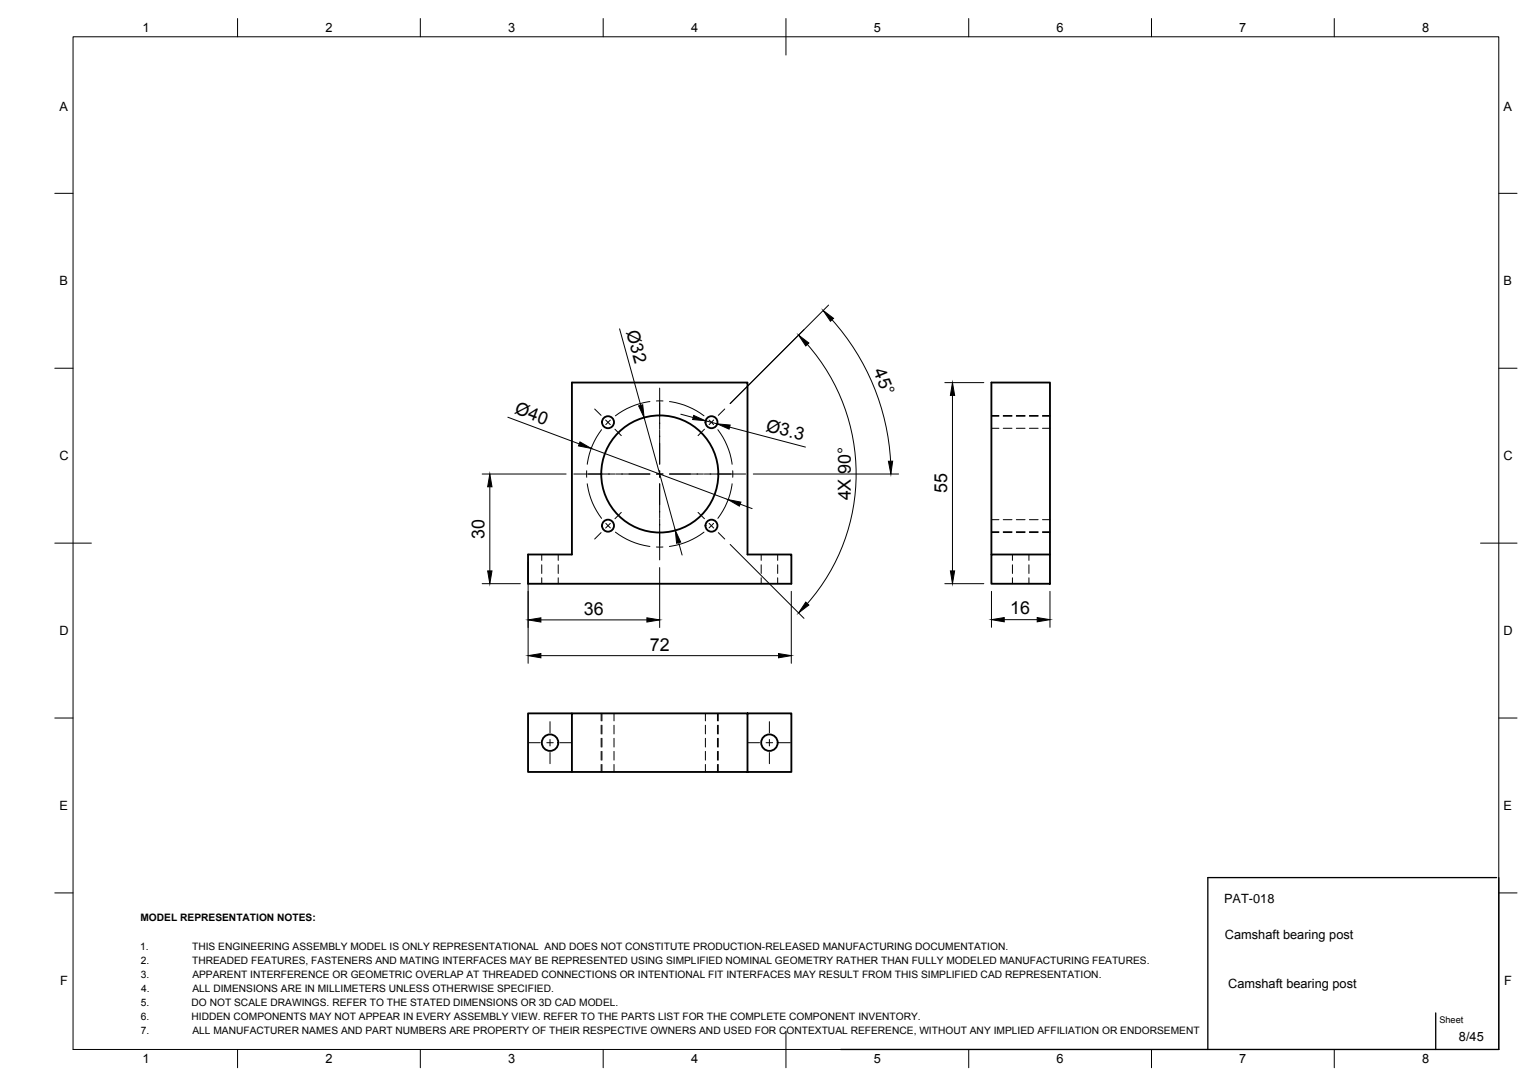
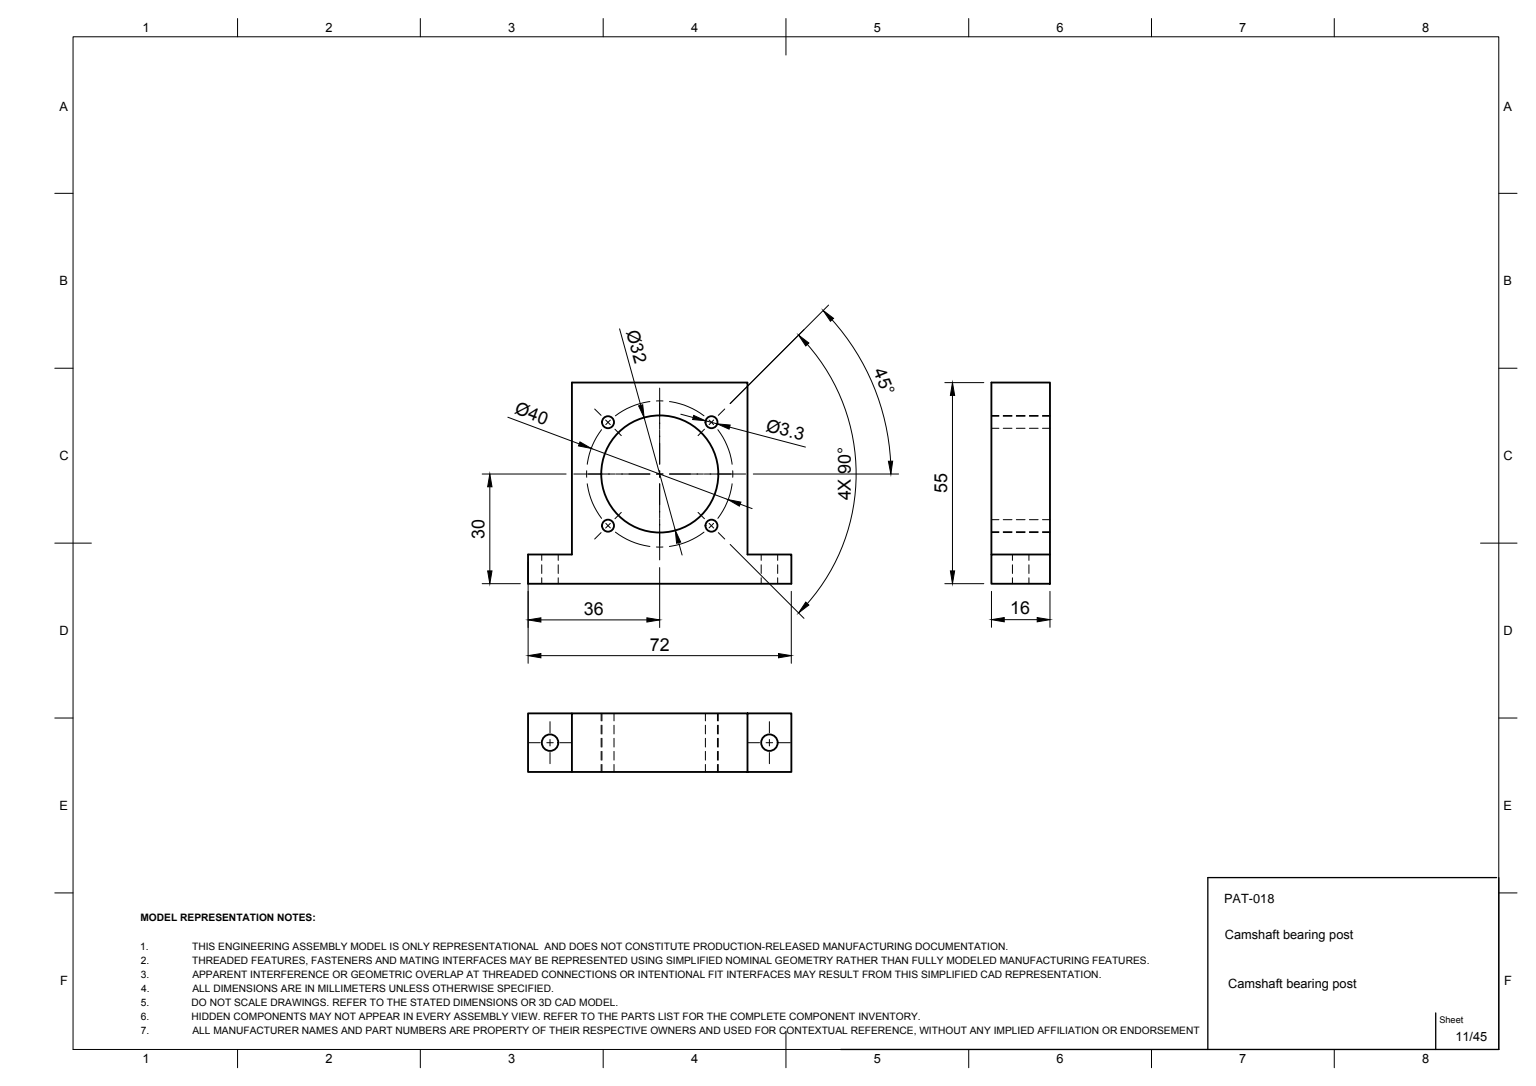
ISO-10303-21;
HEADER;
/* Generated by software containing ST-Developer
 * from STEP Tools, Inc. (www.steptools.com) 
 */

FILE_DESCRIPTION(
/* description */ ('Cam-driven reciprocating slide'),
/* implementation_level */ '2;1');

FILE_NAME(
/* name */ 'Camshaft bearing post.step',
/* time_stamp */ '2026-10-28T03:25:20-07:00',
/* author */ (''),
/* organization */ (''),
/* preprocessor_version */ 'ST-DEVELOPER v20.2',
/* originating_system */ 'Autodesk Translation Framework v15.17.0.0',
/* authorisation */ '');

FILE_SCHEMA (('AUTOMOTIVE_DESIGN { 1 0 10303 214 3 1 1 }'));
ENDSEC;

DATA;
#10=MECHANICAL_DESIGN_GEOMETRIC_PRESENTATION_REPRESENTATION('',(#425),#13277);
#351=SHAPE_REPRESENTATION_RELATIONSHIP('SRR','None',#13444,#388);
#388=ADVANCED_BREP_SHAPE_REPRESENTATION('',(#469),#13239);
#425=STYLED_ITEM('',(#13720),#469);
#469=MANIFOLD_SOLID_BREP('Body1',#6401);
#520=FACE_BOUND('',#1330,.T.);
#521=FACE_BOUND('',#1332,.T.);
#522=FACE_BOUND('',#1336,.T.);
#523=FACE_BOUND('',#1337,.T.);
#524=FACE_BOUND('',#1338,.T.);
#525=FACE_BOUND('',#1339,.T.);
#526=FACE_BOUND('',#1340,.T.);
#527=FACE_BOUND('',#1343,.T.);
#528=FACE_BOUND('',#1344,.T.);
#529=FACE_BOUND('',#1345,.T.);
#530=FACE_BOUND('',#1346,.T.);
#531=FACE_BOUND('',#1347,.T.);
#532=FACE_BOUND('',#1351,.T.);
#533=FACE_BOUND('',#1352,.T.);
#704=PLANE('',#6921);
#705=PLANE('',#6922);
#706=PLANE('',#6923);
#707=PLANE('',#6924);
#708=PLANE('',#6925);
#709=PLANE('',#6926);
#710=PLANE('',#6927);
#711=PLANE('',#6928);
#712=PLANE('',#6929);
#713=PLANE('',#6930);
#930=FACE_OUTER_BOUND('',#1322,.T.);
#931=FACE_OUTER_BOUND('',#1323,.T.);
#932=FACE_OUTER_BOUND('',#1324,.T.);
#933=FACE_OUTER_BOUND('',#1325,.T.);
#934=FACE_OUTER_BOUND('',#1326,.T.);
#935=FACE_OUTER_BOUND('',#1327,.T.);
#936=FACE_OUTER_BOUND('',#1328,.T.);
#937=FACE_OUTER_BOUND('',#1329,.T.);
#938=FACE_OUTER_BOUND('',#1331,.T.);
#939=FACE_OUTER_BOUND('',#1333,.T.);
#940=FACE_OUTER_BOUND('',#1334,.T.);
#941=FACE_OUTER_BOUND('',#1335,.T.);
#942=FACE_OUTER_BOUND('',#1341,.T.);
#943=FACE_OUTER_BOUND('',#1342,.T.);
#944=FACE_OUTER_BOUND('',#1348,.T.);
#945=FACE_OUTER_BOUND('',#1349,.T.);
#946=FACE_OUTER_BOUND('',#1350,.T.);
#1322=EDGE_LOOP('',(#4468,#4469,#4470,#4471));
#1323=EDGE_LOOP('',(#4472,#4473,#4474,#4475));
#1324=EDGE_LOOP('',(#4476,#4477,#4478,#4479));
#1325=EDGE_LOOP('',(#4480,#4481,#4482,#4483));
#1326=EDGE_LOOP('',(#4484,#4485,#4486,#4487));
#1327=EDGE_LOOP('',(#4488,#4489,#4490,#4491));
#1328=EDGE_LOOP('',(#4492,#4493,#4494,#4495));
#1329=EDGE_LOOP('',(#4496,#4497,#4498,#4499));
#1330=EDGE_LOOP('',(#4500));
#1331=EDGE_LOOP('',(#4501,#4502,#4503,#4504));
#1332=EDGE_LOOP('',(#4505));
#1333=EDGE_LOOP('',(#4506,#4507,#4508,#4509));
#1334=EDGE_LOOP('',(#4510,#4511,#4512,#4513));
#1335=EDGE_LOOP('',(#4514,#4515,#4516,#4517,#4518,#4519,#4520,#4521));
#1336=EDGE_LOOP('',(#4522));
#1337=EDGE_LOOP('',(#4523));
#1338=EDGE_LOOP('',(#4524));
#1339=EDGE_LOOP('',(#4525));
#1340=EDGE_LOOP('',(#4526));
#1341=EDGE_LOOP('',(#4527,#4528,#4529,#4530));
#1342=EDGE_LOOP('',(#4531,#4532,#4533,#4534,#4535,#4536,#4537,#4538));
#1343=EDGE_LOOP('',(#4539));
#1344=EDGE_LOOP('',(#4540));
#1345=EDGE_LOOP('',(#4541));
#1346=EDGE_LOOP('',(#4542));
#1347=EDGE_LOOP('',(#4543));
#1348=EDGE_LOOP('',(#4544,#4545,#4546,#4547));
#1349=EDGE_LOOP('',(#4548,#4549,#4550,#4551));
#1350=EDGE_LOOP('',(#4552,#4553,#4554,#4555));
#1351=EDGE_LOOP('',(#4556));
#1352=EDGE_LOOP('',(#4557));
#1887=LINE('',#9889,#2326);
#1888=LINE('',#9895,#2327);
#1889=LINE('',#9901,#2328);
#1890=LINE('',#9907,#2329);
#1891=LINE('',#9913,#2330);
#1892=LINE('',#9919,#2331);
#1893=LINE('',#9925,#2332);
#1894=LINE('',#9930,#2333);
#1895=LINE('',#9932,#2334);
#1896=LINE('',#9934,#2335);
#1897=LINE('',#9935,#2336);
#1898=LINE('',#9939,#2337);
#1899=LINE('',#9941,#2338);
#1900=LINE('',#9943,#2339);
#1901=LINE('',#9944,#2340);
#1902=LINE('',#9947,#2341);
#1903=LINE('',#9949,#2342);
#1904=LINE('',#9950,#2343);
#1905=LINE('',#9953,#2344);
#1906=LINE('',#9955,#2345);
#1907=LINE('',#9956,#2346);
#1908=LINE('',#9959,#2347);
#1909=LINE('',#9961,#2348);
#1910=LINE('',#9962,#2349);
#1911=LINE('',#9963,#2350);
#1912=LINE('',#9966,#2351);
#1913=LINE('',#9967,#2352);
#1914=LINE('',#9970,#2353);
#1915=LINE('',#9971,#2354);
#1916=LINE('',#9972,#2355);
#1917=LINE('',#9974,#2356);
#2326=VECTOR('',#7821,0.225);
#2327=VECTOR('',#7828,0.225);
#2328=VECTOR('',#7835,0.165);
#2329=VECTOR('',#7842,0.165);
#2330=VECTOR('',#7849,0.165);
#2331=VECTOR('',#7856,0.165);
#2332=VECTOR('',#7863,1.6);
#2333=VECTOR('',#7868,1.);
#2334=VECTOR('',#7869,1.);
#2335=VECTOR('',#7870,1.);
#2336=VECTOR('',#7871,1.);
#2337=VECTOR('',#7874,1.);
#2338=VECTOR('',#7875,1.);
#2339=VECTOR('',#7876,1.);
#2340=VECTOR('',#7877,1.);
#2341=VECTOR('',#7880,1.);
#2342=VECTOR('',#7881,1.);
#2343=VECTOR('',#7882,1.);
#2344=VECTOR('',#7885,1.);
#2345=VECTOR('',#7886,1.);
#2346=VECTOR('',#7887,1.);
#2347=VECTOR('',#7890,1.);
#2348=VECTOR('',#7891,1.);
#2349=VECTOR('',#7892,1.);
#2350=VECTOR('',#7893,1.);
#2351=VECTOR('',#7896,1.);
#2352=VECTOR('',#7897,1.);
#2353=VECTOR('',#7900,1.);
#2354=VECTOR('',#7901,1.);
#2355=VECTOR('',#7902,1.);
#2356=VECTOR('',#7905,1.);
#2723=CIRCLE('',#6901,0.225);
#2724=CIRCLE('',#6902,0.225);
#2725=CIRCLE('',#6904,0.225);
#2726=CIRCLE('',#6905,0.225);
#2727=CIRCLE('',#6907,0.165);
#2728=CIRCLE('',#6908,0.165);
#2729=CIRCLE('',#6910,0.165);
#2730=CIRCLE('',#6911,0.165);
#2731=CIRCLE('',#6913,0.165);
#2732=CIRCLE('',#6914,0.165);
#2733=CIRCLE('',#6916,0.165);
#2734=CIRCLE('',#6917,0.165);
#2735=CIRCLE('',#6919,1.6);
#2736=CIRCLE('',#6920,1.6);
#3079=VERTEX_POINT('',#9886);
#3080=VERTEX_POINT('',#9888);
#3081=VERTEX_POINT('',#9892);
#3082=VERTEX_POINT('',#9894);
#3083=VERTEX_POINT('',#9898);
#3084=VERTEX_POINT('',#9900);
#3085=VERTEX_POINT('',#9904);
#3086=VERTEX_POINT('',#9906);
#3087=VERTEX_POINT('',#9910);
#3088=VERTEX_POINT('',#9912);
#3089=VERTEX_POINT('',#9916);
#3090=VERTEX_POINT('',#9918);
#3091=VERTEX_POINT('',#9922);
#3092=VERTEX_POINT('',#9924);
#3093=VERTEX_POINT('',#9928);
#3094=VERTEX_POINT('',#9929);
#3095=VERTEX_POINT('',#9931);
#3096=VERTEX_POINT('',#9933);
#3097=VERTEX_POINT('',#9937);
#3098=VERTEX_POINT('',#9938);
#3099=VERTEX_POINT('',#9940);
#3100=VERTEX_POINT('',#9942);
#3101=VERTEX_POINT('',#9946);
#3102=VERTEX_POINT('',#9948);
#3103=VERTEX_POINT('',#9952);
#3104=VERTEX_POINT('',#9954);
#3105=VERTEX_POINT('',#9958);
#3106=VERTEX_POINT('',#9960);
#3107=VERTEX_POINT('',#9965);
#3108=VERTEX_POINT('',#9969);
#3624=EDGE_CURVE('',#3079,#3079,#2723,.T.);
#3625=EDGE_CURVE('',#3079,#3080,#1887,.T.);
#3626=EDGE_CURVE('',#3080,#3080,#2724,.T.);
#3627=EDGE_CURVE('',#3081,#3081,#2725,.T.);
#3628=EDGE_CURVE('',#3081,#3082,#1888,.T.);
#3629=EDGE_CURVE('',#3082,#3082,#2726,.T.);
#3630=EDGE_CURVE('',#3083,#3083,#2727,.T.);
#3631=EDGE_CURVE('',#3083,#3084,#1889,.T.);
#3632=EDGE_CURVE('',#3084,#3084,#2728,.T.);
#3633=EDGE_CURVE('',#3085,#3085,#2729,.T.);
#3634=EDGE_CURVE('',#3085,#3086,#1890,.T.);
#3635=EDGE_CURVE('',#3086,#3086,#2730,.T.);
#3636=EDGE_CURVE('',#3087,#3087,#2731,.T.);
#3637=EDGE_CURVE('',#3087,#3088,#1891,.T.);
#3638=EDGE_CURVE('',#3088,#3088,#2732,.T.);
#3639=EDGE_CURVE('',#3089,#3089,#2733,.T.);
#3640=EDGE_CURVE('',#3089,#3090,#1892,.T.);
#3641=EDGE_CURVE('',#3090,#3090,#2734,.T.);
#3642=EDGE_CURVE('',#3091,#3091,#2735,.T.);
#3643=EDGE_CURVE('',#3091,#3092,#1893,.T.);
#3644=EDGE_CURVE('',#3092,#3092,#2736,.T.);
#3645=EDGE_CURVE('',#3093,#3094,#1894,.T.);
#3646=EDGE_CURVE('',#3095,#3093,#1895,.T.);
#3647=EDGE_CURVE('',#3095,#3096,#1896,.T.);
#3648=EDGE_CURVE('',#3094,#3096,#1897,.T.);
#3649=EDGE_CURVE('',#3097,#3098,#1898,.T.);
#3650=EDGE_CURVE('',#3099,#3097,#1899,.T.);
#3651=EDGE_CURVE('',#3100,#3099,#1900,.T.);
#3652=EDGE_CURVE('',#3098,#3100,#1901,.T.);
#3653=EDGE_CURVE('',#3100,#3101,#1902,.T.);
#3654=EDGE_CURVE('',#3102,#3099,#1903,.T.);
#3655=EDGE_CURVE('',#3101,#3102,#1904,.T.);
#3656=EDGE_CURVE('',#3103,#3095,#1905,.T.);
#3657=EDGE_CURVE('',#3103,#3104,#1906,.T.);
#3658=EDGE_CURVE('',#3096,#3104,#1907,.T.);
#3659=EDGE_CURVE('',#3093,#3105,#1908,.T.);
#3660=EDGE_CURVE('',#3106,#3105,#1909,.T.);
#3661=EDGE_CURVE('',#3098,#3106,#1910,.T.);
#3662=EDGE_CURVE('',#3101,#3103,#1911,.T.);
#3663=EDGE_CURVE('',#3094,#3107,#1912,.T.);
#3664=EDGE_CURVE('',#3105,#3107,#1913,.T.);
#3665=EDGE_CURVE('',#3097,#3108,#1914,.T.);
#3666=EDGE_CURVE('',#3107,#3108,#1915,.T.);
#3667=EDGE_CURVE('',#3104,#3102,#1916,.T.);
#3668=EDGE_CURVE('',#3108,#3106,#1917,.T.);
#4468=ORIENTED_EDGE('',*,*,#3624,.F.);
#4469=ORIENTED_EDGE('',*,*,#3625,.T.);
#4470=ORIENTED_EDGE('',*,*,#3626,.F.);
#4471=ORIENTED_EDGE('',*,*,#3625,.F.);
#4472=ORIENTED_EDGE('',*,*,#3627,.F.);
#4473=ORIENTED_EDGE('',*,*,#3628,.T.);
#4474=ORIENTED_EDGE('',*,*,#3629,.F.);
#4475=ORIENTED_EDGE('',*,*,#3628,.F.);
#4476=ORIENTED_EDGE('',*,*,#3630,.F.);
#4477=ORIENTED_EDGE('',*,*,#3631,.T.);
#4478=ORIENTED_EDGE('',*,*,#3632,.F.);
#4479=ORIENTED_EDGE('',*,*,#3631,.F.);
#4480=ORIENTED_EDGE('',*,*,#3633,.F.);
#4481=ORIENTED_EDGE('',*,*,#3634,.T.);
#4482=ORIENTED_EDGE('',*,*,#3635,.F.);
#4483=ORIENTED_EDGE('',*,*,#3634,.F.);
#4484=ORIENTED_EDGE('',*,*,#3636,.F.);
#4485=ORIENTED_EDGE('',*,*,#3637,.T.);
#4486=ORIENTED_EDGE('',*,*,#3638,.F.);
#4487=ORIENTED_EDGE('',*,*,#3637,.F.);
#4488=ORIENTED_EDGE('',*,*,#3639,.F.);
#4489=ORIENTED_EDGE('',*,*,#3640,.T.);
#4490=ORIENTED_EDGE('',*,*,#3641,.F.);
#4491=ORIENTED_EDGE('',*,*,#3640,.F.);
#4492=ORIENTED_EDGE('',*,*,#3642,.F.);
#4493=ORIENTED_EDGE('',*,*,#3643,.T.);
#4494=ORIENTED_EDGE('',*,*,#3644,.F.);
#4495=ORIENTED_EDGE('',*,*,#3643,.F.);
#4496=ORIENTED_EDGE('',*,*,#3645,.F.);
#4497=ORIENTED_EDGE('',*,*,#3646,.F.);
#4498=ORIENTED_EDGE('',*,*,#3647,.T.);
#4499=ORIENTED_EDGE('',*,*,#3648,.F.);
#4500=ORIENTED_EDGE('',*,*,#3629,.T.);
#4501=ORIENTED_EDGE('',*,*,#3649,.F.);
#4502=ORIENTED_EDGE('',*,*,#3650,.F.);
#4503=ORIENTED_EDGE('',*,*,#3651,.F.);
#4504=ORIENTED_EDGE('',*,*,#3652,.F.);
#4505=ORIENTED_EDGE('',*,*,#3626,.T.);
#4506=ORIENTED_EDGE('',*,*,#3653,.F.);
#4507=ORIENTED_EDGE('',*,*,#3651,.T.);
#4508=ORIENTED_EDGE('',*,*,#3654,.F.);
#4509=ORIENTED_EDGE('',*,*,#3655,.F.);
#4510=ORIENTED_EDGE('',*,*,#3656,.F.);
#4511=ORIENTED_EDGE('',*,*,#3657,.T.);
#4512=ORIENTED_EDGE('',*,*,#3658,.F.);
#4513=ORIENTED_EDGE('',*,*,#3647,.F.);
#4514=ORIENTED_EDGE('',*,*,#3659,.T.);
#4515=ORIENTED_EDGE('',*,*,#3660,.F.);
#4516=ORIENTED_EDGE('',*,*,#3661,.F.);
#4517=ORIENTED_EDGE('',*,*,#3652,.T.);
#4518=ORIENTED_EDGE('',*,*,#3653,.T.);
#4519=ORIENTED_EDGE('',*,*,#3662,.T.);
#4520=ORIENTED_EDGE('',*,*,#3656,.T.);
#4521=ORIENTED_EDGE('',*,*,#3646,.T.);
#4522=ORIENTED_EDGE('',*,*,#3642,.T.);
#4523=ORIENTED_EDGE('',*,*,#3639,.T.);
#4524=ORIENTED_EDGE('',*,*,#3636,.T.);
#4525=ORIENTED_EDGE('',*,*,#3633,.T.);
#4526=ORIENTED_EDGE('',*,*,#3630,.T.);
#4527=ORIENTED_EDGE('',*,*,#3645,.T.);
#4528=ORIENTED_EDGE('',*,*,#3663,.T.);
#4529=ORIENTED_EDGE('',*,*,#3664,.F.);
#4530=ORIENTED_EDGE('',*,*,#3659,.F.);
#4531=ORIENTED_EDGE('',*,*,#3665,.T.);
#4532=ORIENTED_EDGE('',*,*,#3666,.F.);
#4533=ORIENTED_EDGE('',*,*,#3663,.F.);
#4534=ORIENTED_EDGE('',*,*,#3648,.T.);
#4535=ORIENTED_EDGE('',*,*,#3658,.T.);
#4536=ORIENTED_EDGE('',*,*,#3667,.T.);
#4537=ORIENTED_EDGE('',*,*,#3654,.T.);
#4538=ORIENTED_EDGE('',*,*,#3650,.T.);
#4539=ORIENTED_EDGE('',*,*,#3644,.T.);
#4540=ORIENTED_EDGE('',*,*,#3641,.T.);
#4541=ORIENTED_EDGE('',*,*,#3638,.T.);
#4542=ORIENTED_EDGE('',*,*,#3635,.T.);
#4543=ORIENTED_EDGE('',*,*,#3632,.T.);
#4544=ORIENTED_EDGE('',*,*,#3649,.T.);
#4545=ORIENTED_EDGE('',*,*,#3661,.T.);
#4546=ORIENTED_EDGE('',*,*,#3668,.F.);
#4547=ORIENTED_EDGE('',*,*,#3665,.F.);
#4548=ORIENTED_EDGE('',*,*,#3668,.T.);
#4549=ORIENTED_EDGE('',*,*,#3660,.T.);
#4550=ORIENTED_EDGE('',*,*,#3664,.T.);
#4551=ORIENTED_EDGE('',*,*,#3666,.T.);
#4552=ORIENTED_EDGE('',*,*,#3667,.F.);
#4553=ORIENTED_EDGE('',*,*,#3657,.F.);
#4554=ORIENTED_EDGE('',*,*,#3662,.F.);
#4555=ORIENTED_EDGE('',*,*,#3655,.T.);
#4556=ORIENTED_EDGE('',*,*,#3624,.T.);
#4557=ORIENTED_EDGE('',*,*,#3627,.T.);
#5898=CYLINDRICAL_SURFACE('',#6900,0.225);
#5899=CYLINDRICAL_SURFACE('',#6903,0.225);
#5900=CYLINDRICAL_SURFACE('',#6906,0.165);
#5901=CYLINDRICAL_SURFACE('',#6909,0.165);
#5902=CYLINDRICAL_SURFACE('',#6912,0.165);
#5903=CYLINDRICAL_SURFACE('',#6915,0.165);
#5904=CYLINDRICAL_SURFACE('',#6918,1.6);
#6048=ADVANCED_FACE('',(#930),#5898,.F.);
#6049=ADVANCED_FACE('',(#931),#5899,.F.);
#6050=ADVANCED_FACE('',(#932),#5900,.F.);
#6051=ADVANCED_FACE('',(#933),#5901,.F.);
#6052=ADVANCED_FACE('',(#934),#5902,.F.);
#6053=ADVANCED_FACE('',(#935),#5903,.F.);
#6054=ADVANCED_FACE('',(#936),#5904,.F.);
#6055=ADVANCED_FACE('',(#937,#520),#704,.T.);
#6056=ADVANCED_FACE('',(#938,#521),#705,.T.);
#6057=ADVANCED_FACE('',(#939),#706,.T.);
#6058=ADVANCED_FACE('',(#940),#707,.T.);
#6059=ADVANCED_FACE('',(#941,#522,#523,#524,#525,#526),#708,.T.);
#6060=ADVANCED_FACE('',(#942),#709,.T.);
#6061=ADVANCED_FACE('',(#943,#527,#528,#529,#530,#531),#710,.T.);
#6062=ADVANCED_FACE('',(#944),#711,.T.);
#6063=ADVANCED_FACE('',(#945),#712,.T.);
#6064=ADVANCED_FACE('',(#946,#532,#533),#713,.F.);
#6401=CLOSED_SHELL('',(#6048,#6049,#6050,#6051,#6052,#6053,#6054,#6055,
#6056,#6057,#6058,#6059,#6060,#6061,#6062,#6063,#6064));
#6899=AXIS2_PLACEMENT_3D('',#9884,#7815,#7816);
#6900=AXIS2_PLACEMENT_3D('',#9885,#7817,#7818);
#6901=AXIS2_PLACEMENT_3D('',#9887,#7819,#7820);
#6902=AXIS2_PLACEMENT_3D('',#9890,#7822,#7823);
#6903=AXIS2_PLACEMENT_3D('',#9891,#7824,#7825);
#6904=AXIS2_PLACEMENT_3D('',#9893,#7826,#7827);
#6905=AXIS2_PLACEMENT_3D('',#9896,#7829,#7830);
#6906=AXIS2_PLACEMENT_3D('',#9897,#7831,#7832);
#6907=AXIS2_PLACEMENT_3D('',#9899,#7833,#7834);
#6908=AXIS2_PLACEMENT_3D('',#9902,#7836,#7837);
#6909=AXIS2_PLACEMENT_3D('',#9903,#7838,#7839);
#6910=AXIS2_PLACEMENT_3D('',#9905,#7840,#7841);
#6911=AXIS2_PLACEMENT_3D('',#9908,#7843,#7844);
#6912=AXIS2_PLACEMENT_3D('',#9909,#7845,#7846);
#6913=AXIS2_PLACEMENT_3D('',#9911,#7847,#7848);
#6914=AXIS2_PLACEMENT_3D('',#9914,#7850,#7851);
#6915=AXIS2_PLACEMENT_3D('',#9915,#7852,#7853);
#6916=AXIS2_PLACEMENT_3D('',#9917,#7854,#7855);
#6917=AXIS2_PLACEMENT_3D('',#9920,#7857,#7858);
#6918=AXIS2_PLACEMENT_3D('',#9921,#7859,#7860);
#6919=AXIS2_PLACEMENT_3D('',#9923,#7861,#7862);
#6920=AXIS2_PLACEMENT_3D('',#9926,#7864,#7865);
#6921=AXIS2_PLACEMENT_3D('',#9927,#7866,#7867);
#6922=AXIS2_PLACEMENT_3D('',#9936,#7872,#7873);
#6923=AXIS2_PLACEMENT_3D('',#9945,#7878,#7879);
#6924=AXIS2_PLACEMENT_3D('',#9951,#7883,#7884);
#6925=AXIS2_PLACEMENT_3D('',#9957,#7888,#7889);
#6926=AXIS2_PLACEMENT_3D('',#9964,#7894,#7895);
#6927=AXIS2_PLACEMENT_3D('',#9968,#7898,#7899);
#6928=AXIS2_PLACEMENT_3D('',#9973,#7903,#7904);
#6929=AXIS2_PLACEMENT_3D('',#9975,#7906,#7907);
#6930=AXIS2_PLACEMENT_3D('',#9976,#7908,#7909);
#7815=DIRECTION('axis',(0.,0.,1.));
#7816=DIRECTION('refdir',(1.,0.,0.));
#7817=DIRECTION('center_axis',(0.,0.,1.));
#7818=DIRECTION('ref_axis',(1.,0.,0.));
#7819=DIRECTION('center_axis',(0.,0.,1.));
#7820=DIRECTION('ref_axis',(1.,0.,0.));
#7821=DIRECTION('',(0.,0.,1.));
#7822=DIRECTION('center_axis',(0.,0.,-1.));
#7823=DIRECTION('ref_axis',(1.,0.,0.));
#7824=DIRECTION('center_axis',(0.,0.,1.));
#7825=DIRECTION('ref_axis',(1.,0.,0.));
#7826=DIRECTION('center_axis',(0.,0.,1.));
#7827=DIRECTION('ref_axis',(1.,0.,0.));
#7828=DIRECTION('',(0.,0.,1.));
#7829=DIRECTION('center_axis',(0.,0.,-1.));
#7830=DIRECTION('ref_axis',(1.,0.,0.));
#7831=DIRECTION('center_axis',(0.,1.,0.));
#7832=DIRECTION('ref_axis',(1.,0.,0.));
#7833=DIRECTION('center_axis',(0.,1.,0.));
#7834=DIRECTION('ref_axis',(1.,0.,0.));
#7835=DIRECTION('',(0.,1.,0.));
#7836=DIRECTION('center_axis',(0.,-1.,0.));
#7837=DIRECTION('ref_axis',(1.,0.,0.));
#7838=DIRECTION('center_axis',(0.,1.,0.));
#7839=DIRECTION('ref_axis',(1.,0.,0.));
#7840=DIRECTION('center_axis',(0.,1.,0.));
#7841=DIRECTION('ref_axis',(1.,0.,0.));
#7842=DIRECTION('',(0.,1.,0.));
#7843=DIRECTION('center_axis',(0.,-1.,0.));
#7844=DIRECTION('ref_axis',(1.,0.,0.));
#7845=DIRECTION('center_axis',(0.,1.,0.));
#7846=DIRECTION('ref_axis',(1.,0.,0.));
#7847=DIRECTION('center_axis',(0.,1.,0.));
#7848=DIRECTION('ref_axis',(1.,0.,0.));
#7849=DIRECTION('',(0.,1.,0.));
#7850=DIRECTION('center_axis',(0.,-1.,0.));
#7851=DIRECTION('ref_axis',(1.,0.,0.));
#7852=DIRECTION('center_axis',(0.,1.,0.));
#7853=DIRECTION('ref_axis',(1.,0.,0.));
#7854=DIRECTION('center_axis',(0.,1.,0.));
#7855=DIRECTION('ref_axis',(1.,0.,0.));
#7856=DIRECTION('',(0.,1.,0.));
#7857=DIRECTION('center_axis',(0.,-1.,0.));
#7858=DIRECTION('ref_axis',(1.,0.,0.));
#7859=DIRECTION('center_axis',(0.,1.,0.));
#7860=DIRECTION('ref_axis',(1.,0.,0.));
#7861=DIRECTION('center_axis',(0.,1.,0.));
#7862=DIRECTION('ref_axis',(1.,0.,0.));
#7863=DIRECTION('',(0.,1.,0.));
#7864=DIRECTION('center_axis',(0.,-1.,0.));
#7865=DIRECTION('ref_axis',(1.,0.,0.));
#7866=DIRECTION('center_axis',(0.,0.,1.));
#7867=DIRECTION('ref_axis',(1.,0.,0.));
#7868=DIRECTION('',(0.,1.,0.));
#7869=DIRECTION('',(-1.,0.,0.));
#7870=DIRECTION('',(0.,1.,0.));
#7871=DIRECTION('',(1.,0.,0.));
#7872=DIRECTION('center_axis',(0.,0.,1.));
#7873=DIRECTION('ref_axis',(1.,0.,0.));
#7874=DIRECTION('',(0.,-1.,0.));
#7875=DIRECTION('',(1.,0.,0.));
#7876=DIRECTION('',(0.,1.,0.));
#7877=DIRECTION('',(-1.,0.,0.));
#7878=DIRECTION('center_axis',(-1.,0.,0.));
#7879=DIRECTION('ref_axis',(0.,0.,1.));
#7880=DIRECTION('',(0.,0.,-1.));
#7881=DIRECTION('',(0.,0.,1.));
#7882=DIRECTION('',(0.,1.,0.));
#7883=DIRECTION('center_axis',(1.,0.,0.));
#7884=DIRECTION('ref_axis',(0.,0.,-1.));
#7885=DIRECTION('',(0.,0.,1.));
#7886=DIRECTION('',(0.,1.,0.));
#7887=DIRECTION('',(0.,0.,-1.));
#7888=DIRECTION('center_axis',(0.,-1.,0.));
#7889=DIRECTION('ref_axis',(1.,0.,0.));
#7890=DIRECTION('',(0.,0.,1.));
#7891=DIRECTION('',(1.,0.,0.));
#7892=DIRECTION('',(0.,0.,1.));
#7893=DIRECTION('',(1.,0.,0.));
#7894=DIRECTION('center_axis',(1.,0.,0.));
#7895=DIRECTION('ref_axis',(0.,1.,0.));
#7896=DIRECTION('',(0.,0.,1.));
#7897=DIRECTION('',(0.,1.,0.));
#7898=DIRECTION('center_axis',(0.,1.,0.));
#7899=DIRECTION('ref_axis',(-1.,0.,0.));
#7900=DIRECTION('',(0.,0.,1.));
#7901=DIRECTION('',(-1.,0.,0.));
#7902=DIRECTION('',(-1.,0.,0.));
#7903=DIRECTION('center_axis',(-1.,0.,0.));
#7904=DIRECTION('ref_axis',(0.,-1.,0.));
#7905=DIRECTION('',(0.,-1.,0.));
#7906=DIRECTION('center_axis',(0.,0.,1.));
#7907=DIRECTION('ref_axis',(1.,0.,0.));
#7908=DIRECTION('center_axis',(0.,0.,1.));
#7909=DIRECTION('ref_axis',(1.,0.,0.));
#9884=CARTESIAN_POINT('',(0.,0.,0.));
#9885=CARTESIAN_POINT('Origin',(-3.,-2.5,0.9));
#9886=CARTESIAN_POINT('',(-3.225,-2.5,1.));
#9887=CARTESIAN_POINT('Origin',(-3.,-2.5,1.));
#9888=CARTESIAN_POINT('',(-3.225,-2.5,1.8));
#9889=CARTESIAN_POINT('',(-3.225,-2.5,0.9));
#9890=CARTESIAN_POINT('Origin',(-3.,-2.5,1.8));
#9891=CARTESIAN_POINT('Origin',(3.,-2.5,0.9));
#9892=CARTESIAN_POINT('',(2.775,-2.5,1.));
#9893=CARTESIAN_POINT('Origin',(3.,-2.5,1.));
#9894=CARTESIAN_POINT('',(2.775,-2.5,1.8));
#9895=CARTESIAN_POINT('',(2.775,-2.5,0.9));
#9896=CARTESIAN_POINT('Origin',(3.,-2.5,1.8));
#9897=CARTESIAN_POINT('Origin',(-1.4142135623731,-3.4,2.58578643762691));
#9898=CARTESIAN_POINT('',(-1.5792135623731,-3.3,2.58578643762691));
#9899=CARTESIAN_POINT('Origin',(-1.4142135623731,-3.3,2.58578643762691));
#9900=CARTESIAN_POINT('',(-1.5792135623731,-1.7,2.58578643762691));
#9901=CARTESIAN_POINT('',(-1.5792135623731,-3.4,2.58578643762691));
#9902=CARTESIAN_POINT('Origin',(-1.4142135623731,-1.7,2.58578643762691));
#9903=CARTESIAN_POINT('Origin',(-1.41421356237309,-3.4,5.41421356237309));
#9904=CARTESIAN_POINT('',(-1.57921356237309,-3.3,5.41421356237309));
#9905=CARTESIAN_POINT('Origin',(-1.41421356237309,-3.3,5.41421356237309));
#9906=CARTESIAN_POINT('',(-1.57921356237309,-1.7,5.41421356237309));
#9907=CARTESIAN_POINT('',(-1.57921356237309,-3.4,5.41421356237309));
#9908=CARTESIAN_POINT('Origin',(-1.41421356237309,-1.7,5.41421356237309));
#9909=CARTESIAN_POINT('Origin',(1.4142135623731,-3.4,5.41421356237309));
#9910=CARTESIAN_POINT('',(1.2492135623731,-3.3,5.41421356237309));
#9911=CARTESIAN_POINT('Origin',(1.4142135623731,-3.3,5.41421356237309));
#9912=CARTESIAN_POINT('',(1.2492135623731,-1.7,5.41421356237309));
#9913=CARTESIAN_POINT('',(1.2492135623731,-3.4,5.41421356237309));
#9914=CARTESIAN_POINT('Origin',(1.4142135623731,-1.7,5.41421356237309));
#9915=CARTESIAN_POINT('Origin',(1.41421356237309,-3.4,2.5857864376269));
#9916=CARTESIAN_POINT('',(1.24921356237309,-3.3,2.5857864376269));
#9917=CARTESIAN_POINT('Origin',(1.41421356237309,-3.3,2.5857864376269));
#9918=CARTESIAN_POINT('',(1.24921356237309,-1.7,2.5857864376269));
#9919=CARTESIAN_POINT('',(1.24921356237309,-3.4,2.5857864376269));
#9920=CARTESIAN_POINT('Origin',(1.41421356237309,-1.7,2.5857864376269));
#9921=CARTESIAN_POINT('Origin',(0.,-3.4,4.));
#9922=CARTESIAN_POINT('',(-1.6,-3.3,4.));
#9923=CARTESIAN_POINT('Origin',(0.,-3.3,4.));
#9924=CARTESIAN_POINT('',(-1.6,-1.7,4.));
#9925=CARTESIAN_POINT('',(-1.6,-3.4,4.));
#9926=CARTESIAN_POINT('Origin',(0.,-1.7,4.));
#9927=CARTESIAN_POINT('Origin',(-3.6,-3.3,1.8));
#9928=CARTESIAN_POINT('',(2.4,-3.3,1.8));
#9929=CARTESIAN_POINT('',(2.4,-1.7,1.8));
#9930=CARTESIAN_POINT('',(2.4,-3.3,1.8));
#9931=CARTESIAN_POINT('',(3.6,-3.3,1.8));
#9932=CARTESIAN_POINT('',(3.6,-3.3,1.8));
#9933=CARTESIAN_POINT('',(3.6,-1.7,1.8));
#9934=CARTESIAN_POINT('',(3.6,-3.3,1.8));
#9935=CARTESIAN_POINT('',(3.6,-1.7,1.8));
#9936=CARTESIAN_POINT('Origin',(-3.6,-3.3,1.8));
#9937=CARTESIAN_POINT('',(-2.4,-1.7,1.8));
#9938=CARTESIAN_POINT('',(-2.4,-3.3,1.8));
#9939=CARTESIAN_POINT('',(-2.4,-2.5,1.8));
#9940=CARTESIAN_POINT('',(-3.6,-1.7,1.8));
#9941=CARTESIAN_POINT('',(3.6,-1.7,1.8));
#9942=CARTESIAN_POINT('',(-3.6,-3.3,1.8));
#9943=CARTESIAN_POINT('',(-3.6,-3.3,1.8));
#9944=CARTESIAN_POINT('',(3.6,-3.3,1.8));
#9945=CARTESIAN_POINT('Origin',(-3.6,-3.3,1.));
#9946=CARTESIAN_POINT('',(-3.6,-3.3,1.));
#9947=CARTESIAN_POINT('',(-3.6,-3.3,1.8));
#9948=CARTESIAN_POINT('',(-3.6,-1.7,1.));
#9949=CARTESIAN_POINT('',(-3.6,-1.7,1.8));
#9950=CARTESIAN_POINT('',(-3.6,-3.3,1.));
#9951=CARTESIAN_POINT('Origin',(3.6,-3.3,1.8));
#9952=CARTESIAN_POINT('',(3.6,-3.3,1.));
#9953=CARTESIAN_POINT('',(3.6,-3.3,1.));
#9954=CARTESIAN_POINT('',(3.6,-1.7,1.));
#9955=CARTESIAN_POINT('',(3.6,-3.3,1.));
#9956=CARTESIAN_POINT('',(3.6,-1.7,1.));
#9957=CARTESIAN_POINT('Origin',(-2.4,-3.3,1.));
#9958=CARTESIAN_POINT('',(2.4,-3.3,6.5));
#9959=CARTESIAN_POINT('',(2.4,-3.3,1.));
#9960=CARTESIAN_POINT('',(-2.4,-3.3,6.5));
#9961=CARTESIAN_POINT('',(-2.4,-3.3,6.5));
#9962=CARTESIAN_POINT('',(-2.4,-3.3,1.));
#9963=CARTESIAN_POINT('',(-3.6,-3.3,1.));
#9964=CARTESIAN_POINT('Origin',(2.4,-3.3,1.));
#9965=CARTESIAN_POINT('',(2.4,-1.7,6.5));
#9966=CARTESIAN_POINT('',(2.4,-1.7,1.));
#9967=CARTESIAN_POINT('',(2.4,-3.3,6.5));
#9968=CARTESIAN_POINT('Origin',(2.4,-1.7,1.));
#9969=CARTESIAN_POINT('',(-2.4,-1.7,6.5));
#9970=CARTESIAN_POINT('',(-2.4,-1.7,1.));
#9971=CARTESIAN_POINT('',(2.4,-1.7,6.5));
#9972=CARTESIAN_POINT('',(-3.6,-1.7,1.));
#9973=CARTESIAN_POINT('Origin',(-2.4,-1.7,1.));
#9974=CARTESIAN_POINT('',(-2.4,-1.7,6.5));
#9975=CARTESIAN_POINT('Origin',(0.,-2.5,6.5));
#9976=CARTESIAN_POINT('Origin',(0.,-2.5,1.));
#13195=UNCERTAINTY_MEASURE_WITH_UNIT(LENGTH_MEASURE(0.001),#13278,
'DISTANCE_ACCURACY_VALUE',
'Maximum model space distance between geometric entities at asserted c
onnectivities');
#13233=UNCERTAINTY_MEASURE_WITH_UNIT(LENGTH_MEASURE(0.001),#13278,
'DISTANCE_ACCURACY_VALUE',
'Maximum model space distance between geometric entities at asserted c
onnectivities');
#13239=(
GEOMETRIC_REPRESENTATION_CONTEXT(3)
GLOBAL_UNCERTAINTY_ASSIGNED_CONTEXT((#13195))
GLOBAL_UNIT_ASSIGNED_CONTEXT((#13278,#13280,#13281))
REPRESENTATION_CONTEXT('','3D')
);
#13277=(
GEOMETRIC_REPRESENTATION_CONTEXT(3)
GLOBAL_UNCERTAINTY_ASSIGNED_CONTEXT((#13233))
GLOBAL_UNIT_ASSIGNED_CONTEXT((#13278,#13280,#13281))
REPRESENTATION_CONTEXT('','3D')
);
#13278=(
LENGTH_UNIT()
NAMED_UNIT(*)
SI_UNIT(.CENTI.,.METRE.)
);
#13280=(
NAMED_UNIT(*)
PLANE_ANGLE_UNIT()
SI_UNIT($,.RADIAN.)
);
#13281=(
NAMED_UNIT(*)
SI_UNIT($,.STERADIAN.)
SOLID_ANGLE_UNIT()
);
#13287=SHAPE_DEFINITION_REPRESENTATION(#13330,#13444);
#13330=PRODUCT_DEFINITION_SHAPE('',$,#13488);
#13444=SHAPE_REPRESENTATION('',(#6899),#13239);
#13482=PRODUCT_DEFINITION_CONTEXT('part definition',#13613,'design');
#13488=PRODUCT_DEFINITION('Camshaft bearing post',
'Camshaft bearing post',#13531,#13482);
#13531=PRODUCT_DEFINITION_FORMATION('',$,#13620);
#13613=APPLICATION_CONTEXT(
'Core Data for Automotive Mechanical Design Process');
#13614=PRODUCT_CONTEXT('part definition',#13613,'mechanical');
#13620=PRODUCT('Camshaft bearing post','Camshaft bearing post',
'Camshaft bearing post',(#13614));
#13714=COLOUR_RGB('Grey',0.48,0.52,0.57);
#13715=FILL_AREA_STYLE_COLOUR('',#13714);
#13716=FILL_AREA_STYLE('',(#13715));
#13717=SURFACE_STYLE_FILL_AREA(#13716);
#13718=SURFACE_SIDE_STYLE('',(#13717));
#13719=SURFACE_STYLE_USAGE(.BOTH.,#13718);
#13720=PRESENTATION_STYLE_ASSIGNMENT((#13719));
ENDSEC;
END-ISO-10303-21;
